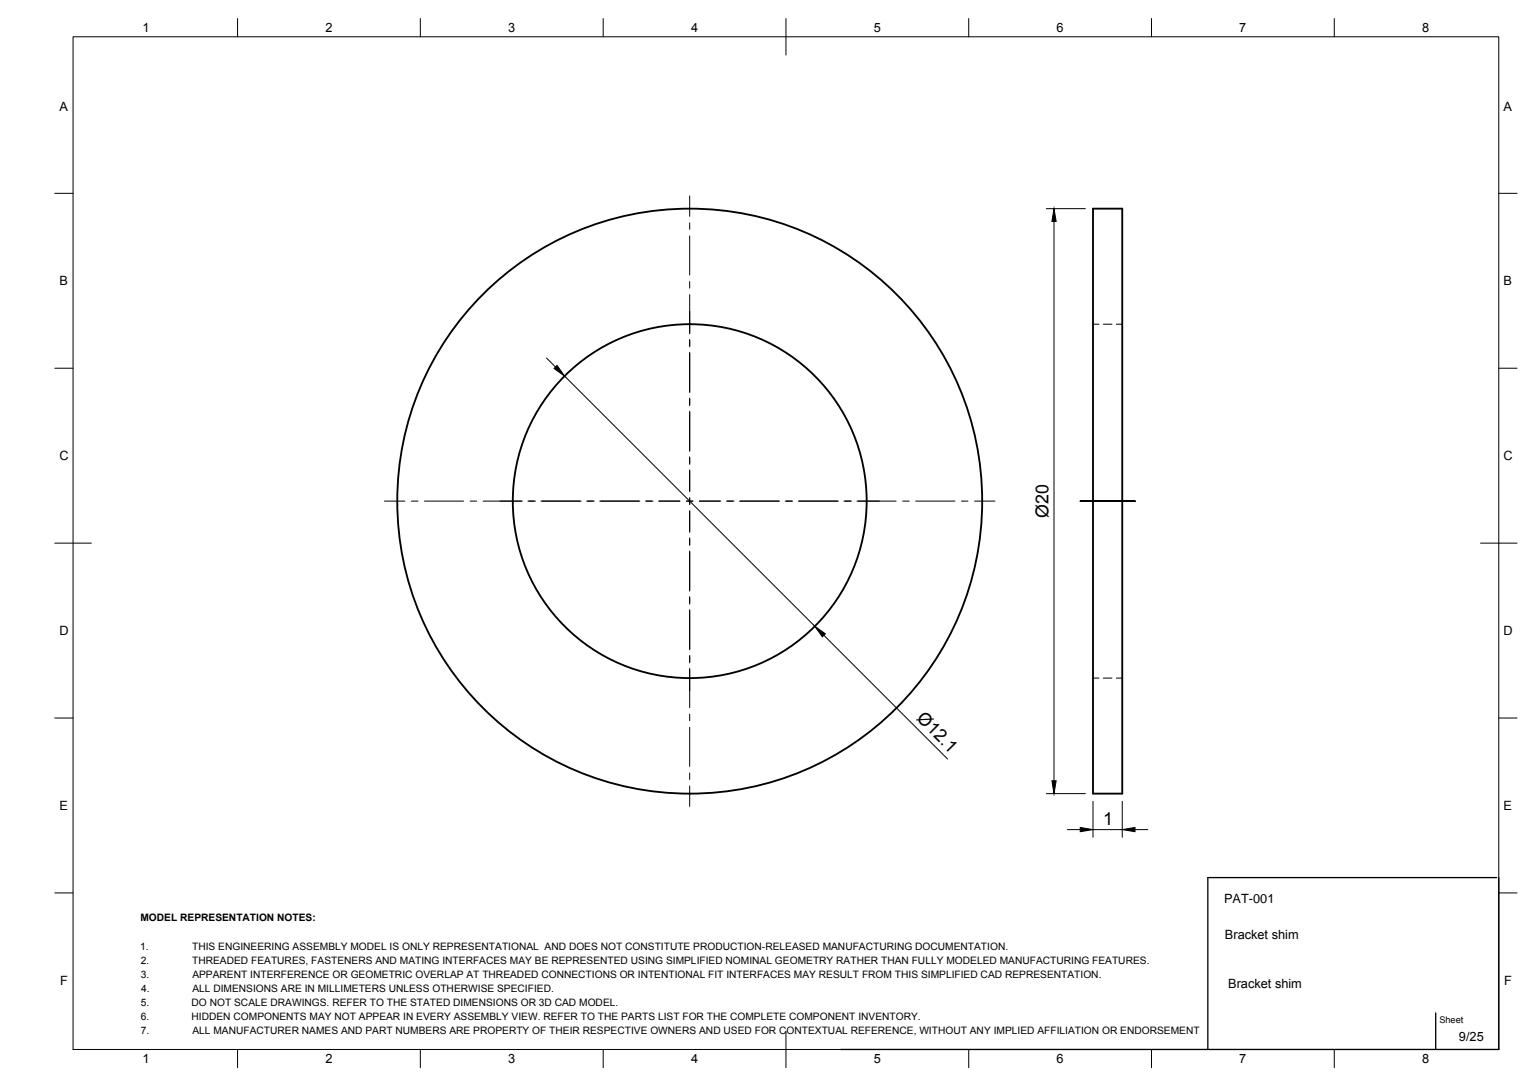
ISO-10303-21;
HEADER;
/* Generated by software containing ST-Developer
 * from STEP Tools, Inc. (www.steptools.com) 
 */

FILE_DESCRIPTION(
/* description */ ('PAT-001'),
/* implementation_level */ '2;1');

FILE_NAME(
/* name */ 'Bracket shim.step',
/* time_stamp */ '2026-10-29T17:07:15-07:00',
/* author */ (''),
/* organization */ (''),
/* preprocessor_version */ 'ST-DEVELOPER v20.2',
/* originating_system */ 'Autodesk Translation Framework v15.17.0.0',
/* authorisation */ '');

FILE_SCHEMA (('AUTOMOTIVE_DESIGN { 1 0 10303 214 3 1 1 }'));
ENDSEC;

DATA;
#10=MECHANICAL_DESIGN_GEOMETRIC_PRESENTATION_REPRESENTATION('',(#377),#9622);
#327=SHAPE_REPRESENTATION_RELATIONSHIP('SRR','None',#9750,#352);
#352=ADVANCED_BREP_SHAPE_REPRESENTATION('',(#410),#9599);
#377=STYLED_ITEM('',(#9941),#410);
#410=MANIFOLD_SOLID_BREP('Body1',#5202);
#447=FACE_BOUND('',#1047,.T.);
#448=FACE_BOUND('',#1049,.T.);
#540=PLANE('',#5567);
#541=PLANE('',#5568);
#738=FACE_OUTER_BOUND('',#1044,.T.);
#739=FACE_OUTER_BOUND('',#1045,.T.);
#740=FACE_OUTER_BOUND('',#1046,.T.);
#741=FACE_OUTER_BOUND('',#1048,.T.);
#1044=EDGE_LOOP('',(#3583,#3584,#3585,#3586));
#1045=EDGE_LOOP('',(#3587,#3588,#3589,#3590));
#1046=EDGE_LOOP('',(#3591));
#1047=EDGE_LOOP('',(#3592));
#1048=EDGE_LOOP('',(#3593));
#1049=EDGE_LOOP('',(#3594));
#1409=LINE('',#7797,#1814);
#1410=LINE('',#7803,#1815);
#1814=VECTOR('',#6226,0.605);
#1815=VECTOR('',#6233,1.);
#2230=CIRCLE('',#5562,0.605);
#2231=CIRCLE('',#5563,0.605);
#2232=CIRCLE('',#5565,1.);
#2233=CIRCLE('',#5566,1.);
#2442=VERTEX_POINT('',#7794);
#2443=VERTEX_POINT('',#7796);
#2444=VERTEX_POINT('',#7800);
#2445=VERTEX_POINT('',#7802);
#2895=EDGE_CURVE('',#2442,#2442,#2230,.T.);
#2896=EDGE_CURVE('',#2442,#2443,#1409,.T.);
#2897=EDGE_CURVE('',#2443,#2443,#2231,.T.);
#2898=EDGE_CURVE('',#2444,#2444,#2232,.T.);
#2899=EDGE_CURVE('',#2444,#2445,#1410,.T.);
#2900=EDGE_CURVE('',#2445,#2445,#2233,.T.);
#3583=ORIENTED_EDGE('',*,*,#2895,.F.);
#3584=ORIENTED_EDGE('',*,*,#2896,.T.);
#3585=ORIENTED_EDGE('',*,*,#2897,.T.);
#3586=ORIENTED_EDGE('',*,*,#2896,.F.);
#3587=ORIENTED_EDGE('',*,*,#2898,.F.);
#3588=ORIENTED_EDGE('',*,*,#2899,.T.);
#3589=ORIENTED_EDGE('',*,*,#2900,.T.);
#3590=ORIENTED_EDGE('',*,*,#2899,.F.);
#3591=ORIENTED_EDGE('',*,*,#2898,.T.);
#3592=ORIENTED_EDGE('',*,*,#2895,.T.);
#3593=ORIENTED_EDGE('',*,*,#2900,.F.);
#3594=ORIENTED_EDGE('',*,*,#2897,.F.);
#4838=CYLINDRICAL_SURFACE('',#5561,0.605);
#4839=CYLINDRICAL_SURFACE('',#5564,1.);
#4925=ADVANCED_FACE('',(#738),#4838,.F.);
#4926=ADVANCED_FACE('',(#739),#4839,.T.);
#4927=ADVANCED_FACE('',(#740,#447),#540,.T.);
#4928=ADVANCED_FACE('',(#741,#448),#541,.F.);
#5202=CLOSED_SHELL('',(#4925,#4926,#4927,#4928));
#5560=AXIS2_PLACEMENT_3D('',#7792,#6220,#6221);
#5561=AXIS2_PLACEMENT_3D('',#7793,#6222,#6223);
#5562=AXIS2_PLACEMENT_3D('',#7795,#6224,#6225);
#5563=AXIS2_PLACEMENT_3D('',#7798,#6227,#6228);
#5564=AXIS2_PLACEMENT_3D('',#7799,#6229,#6230);
#5565=AXIS2_PLACEMENT_3D('',#7801,#6231,#6232);
#5566=AXIS2_PLACEMENT_3D('',#7804,#6234,#6235);
#5567=AXIS2_PLACEMENT_3D('',#7805,#6236,#6237);
#5568=AXIS2_PLACEMENT_3D('',#7806,#6238,#6239);
#6220=DIRECTION('axis',(0.,0.,1.));
#6221=DIRECTION('refdir',(1.,0.,0.));
#6222=DIRECTION('center_axis',(0.,1.,0.));
#6223=DIRECTION('ref_axis',(1.,0.,0.));
#6224=DIRECTION('center_axis',(0.,-1.,0.));
#6225=DIRECTION('ref_axis',(1.,0.,0.));
#6226=DIRECTION('',(0.,-1.,0.));
#6227=DIRECTION('center_axis',(0.,-1.,0.));
#6228=DIRECTION('ref_axis',(1.,0.,0.));
#6229=DIRECTION('center_axis',(0.,1.,0.));
#6230=DIRECTION('ref_axis',(1.,0.,0.));
#6231=DIRECTION('center_axis',(0.,1.,0.));
#6232=DIRECTION('ref_axis',(1.,0.,0.));
#6233=DIRECTION('',(0.,-1.,0.));
#6234=DIRECTION('center_axis',(0.,1.,0.));
#6235=DIRECTION('ref_axis',(1.,0.,0.));
#6236=DIRECTION('center_axis',(0.,1.,0.));
#6237=DIRECTION('ref_axis',(1.,0.,0.));
#6238=DIRECTION('center_axis',(0.,1.,0.));
#6239=DIRECTION('ref_axis',(1.,0.,0.));
#7792=CARTESIAN_POINT('',(0.,0.,0.));
#7793=CARTESIAN_POINT('Origin',(0.,-2.5,4.5));
#7794=CARTESIAN_POINT('',(-0.605,-2.4,4.5));
#7795=CARTESIAN_POINT('Origin',(0.,-2.4,4.5));
#7796=CARTESIAN_POINT('',(-0.605,-2.5,4.5));
#7797=CARTESIAN_POINT('',(-0.605,-2.5,4.5));
#7798=CARTESIAN_POINT('Origin',(0.,-2.5,4.5));
#7799=CARTESIAN_POINT('Origin',(0.,-2.5,4.5));
#7800=CARTESIAN_POINT('',(-1.,-2.4,4.5));
#7801=CARTESIAN_POINT('Origin',(0.,-2.4,4.5));
#7802=CARTESIAN_POINT('',(-1.,-2.5,4.5));
#7803=CARTESIAN_POINT('',(-1.,-2.5,4.5));
#7804=CARTESIAN_POINT('Origin',(0.,-2.5,4.5));
#7805=CARTESIAN_POINT('Origin',(0.,-2.4,4.5));
#7806=CARTESIAN_POINT('Origin',(0.,-2.5,4.5));
#9569=UNCERTAINTY_MEASURE_WITH_UNIT(LENGTH_MEASURE(0.001),#9623,
'DISTANCE_ACCURACY_VALUE',
'Maximum model space distance between geometric entities at asserted c
onnectivities');
#9592=UNCERTAINTY_MEASURE_WITH_UNIT(LENGTH_MEASURE(0.001),#9623,
'DISTANCE_ACCURACY_VALUE',
'Maximum model space distance between geometric entities at asserted c
onnectivities');
#9599=(
GEOMETRIC_REPRESENTATION_CONTEXT(3)
GLOBAL_UNCERTAINTY_ASSIGNED_CONTEXT((#9569))
GLOBAL_UNIT_ASSIGNED_CONTEXT((#9623,#9625,#9626))
REPRESENTATION_CONTEXT('','3D')
);
#9622=(
GEOMETRIC_REPRESENTATION_CONTEXT(3)
GLOBAL_UNCERTAINTY_ASSIGNED_CONTEXT((#9592))
GLOBAL_UNIT_ASSIGNED_CONTEXT((#9623,#9625,#9626))
REPRESENTATION_CONTEXT('','3D')
);
#9623=(
LENGTH_UNIT()
NAMED_UNIT(*)
SI_UNIT(.CENTI.,.METRE.)
);
#9625=(
NAMED_UNIT(*)
PLANE_ANGLE_UNIT()
SI_UNIT($,.RADIAN.)
);
#9626=(
NAMED_UNIT(*)
SI_UNIT($,.STERADIAN.)
SOLID_ANGLE_UNIT()
);
#9633=SHAPE_DEFINITION_REPRESENTATION(#9662,#9750);
#9662=PRODUCT_DEFINITION_SHAPE('',$,#9780);
#9750=SHAPE_REPRESENTATION('',(#5560),#9599);
#9773=PRODUCT_DEFINITION_CONTEXT('part definition',#9862,'design');
#9780=PRODUCT_DEFINITION('Bracket shim','Bracket shim',#9809,#9773);
#9809=PRODUCT_DEFINITION_FORMATION('',$,#9870);
#9862=APPLICATION_CONTEXT(
'Core Data for Automotive Mechanical Design Process');
#9863=PRODUCT_CONTEXT('part definition',#9862,'mechanical');
#9870=PRODUCT('Bracket shim','Bracket shim','Bracket shim',(#9863));
#9935=COLOUR_RGB('Dark Blue',0.08,0.2,0.34);
#9936=FILL_AREA_STYLE_COLOUR('',#9935);
#9937=FILL_AREA_STYLE('',(#9936));
#9938=SURFACE_STYLE_FILL_AREA(#9937);
#9939=SURFACE_SIDE_STYLE('',(#9938));
#9940=SURFACE_STYLE_USAGE(.BOTH.,#9939);
#9941=PRESENTATION_STYLE_ASSIGNMENT((#9940));
ENDSEC;
END-ISO-10303-21;
